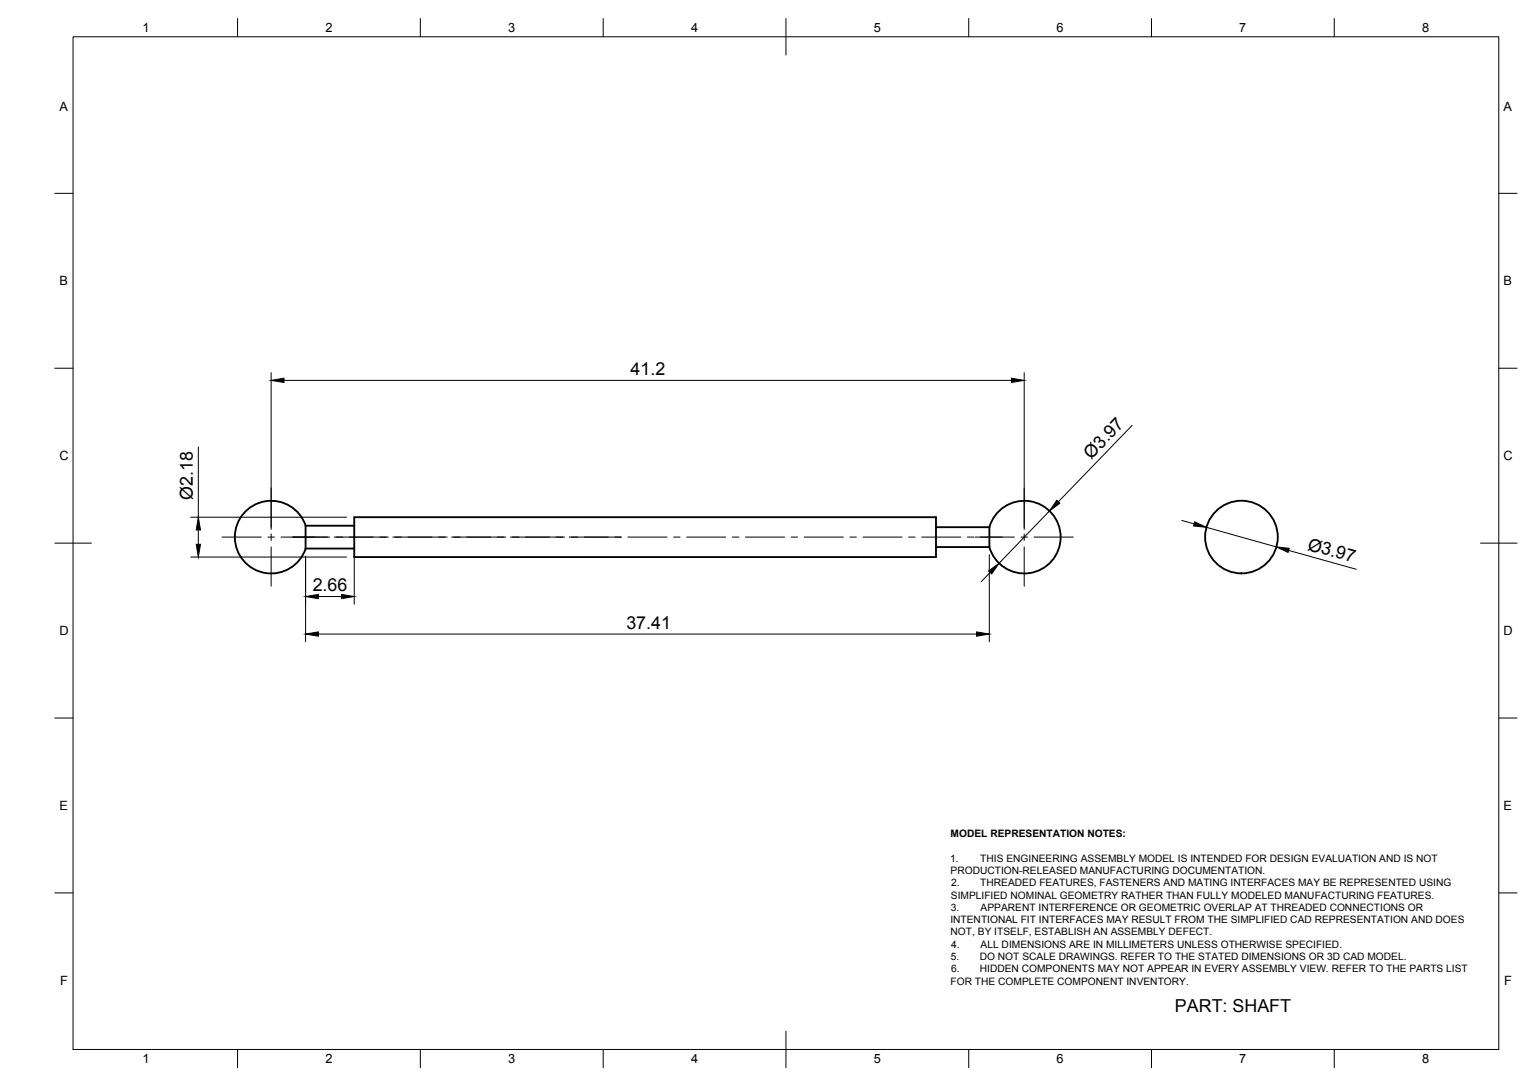
ISO-10303-21;
HEADER;
/* Generated by software containing ST-Developer
 * from STEP Tools, Inc. (www.steptools.com) 
 */

FILE_DESCRIPTION(
/* description */ (''),
/* implementation_level */ '2;1');

FILE_NAME(
/* name */ 'Shaft.step',
/* time_stamp */ '2026-10-04T22:56:18-07:00',
/* author */ (''),
/* organization */ (''),
/* preprocessor_version */ 'ST-DEVELOPER v20.2',
/* originating_system */ 'Autodesk Translation Framework v15.15.0.0',
/* authorisation */ '');

FILE_SCHEMA (('AUTOMOTIVE_DESIGN { 1 0 10303 214 3 1 1 }'));
ENDSEC;

DATA;
#10=MECHANICAL_DESIGN_GEOMETRIC_PRESENTATION_REPRESENTATION('',(#192),#14544);
#169=SPHERICAL_SURFACE('',#1978,1.9854168202488);
#170=SPHERICAL_SURFACE('',#1980,1.9854168202488);
#176=SHAPE_REPRESENTATION_RELATIONSHIP('SRR','None',#14578,#184);
#184=ADVANCED_BREP_SHAPE_REPRESENTATION('',(#200),#14538);
#192=STYLED_ITEM('',(#14627),#200);
#200=MANIFOLD_SOLID_BREP('Body1',#1828);
#215=LINE('',#2670,#271);
#216=LINE('',#2678,#272);
#217=LINE('',#2685,#273);
#271=VECTOR('',#2229,0.544851764215984);
#272=VECTOR('',#2240,1.08970352843197);
#273=VECTOR('',#2249,0.625182919763592);
#327=CYLINDRICAL_SURFACE('',#1967,0.544851764215984);
#328=CYLINDRICAL_SURFACE('',#1972,1.08970352843197);
#329=CYLINDRICAL_SURFACE('',#1976,0.625182919763592);
#378=FACE_BOUND('',#534,.T.);
#379=FACE_BOUND('',#537,.T.);
#419=FACE_OUTER_BOUND('',#532,.T.);
#420=FACE_OUTER_BOUND('',#533,.T.);
#421=FACE_OUTER_BOUND('',#535,.T.);
#422=FACE_OUTER_BOUND('',#536,.T.);
#423=FACE_OUTER_BOUND('',#538,.T.);
#424=FACE_OUTER_BOUND('',#539,.T.);
#425=FACE_OUTER_BOUND('',#540,.T.);
#532=EDGE_LOOP('',(#1229,#1230,#1231,#1232));
#533=EDGE_LOOP('',(#1233));
#534=EDGE_LOOP('',(#1234));
#535=EDGE_LOOP('',(#1235,#1236,#1237,#1238));
#536=EDGE_LOOP('',(#1239));
#537=EDGE_LOOP('',(#1240));
#538=EDGE_LOOP('',(#1241,#1242,#1243,#1244));
#539=EDGE_LOOP('',(#1245,#1246,#1247));
#540=EDGE_LOOP('',(#1248,#1249,#1250));
#658=CIRCLE('',#1968,0.544851764215984);
#659=CIRCLE('',#1969,0.544851764215984);
#660=CIRCLE('',#1971,1.08970352843197);
#661=CIRCLE('',#1973,1.08970352843197);
#662=CIRCLE('',#1975,0.625182919763592);
#663=CIRCLE('',#1977,0.625182919763592);
#664=CIRCLE('',#1979,1.9854168202488);
#665=CIRCLE('',#1981,1.9854168202488);
#744=VERTEX_POINT('',#2667);
#745=VERTEX_POINT('',#2669);
#746=VERTEX_POINT('',#2673);
#747=VERTEX_POINT('',#2676);
#748=VERTEX_POINT('',#2680);
#749=VERTEX_POINT('',#2683);
#750=VERTEX_POINT('',#2687);
#751=VERTEX_POINT('',#2690);
#943=EDGE_CURVE('',#744,#744,#658,.T.);
#944=EDGE_CURVE('',#744,#745,#215,.T.);
#945=EDGE_CURVE('',#745,#745,#659,.T.);
#946=EDGE_CURVE('',#746,#746,#660,.T.);
#947=EDGE_CURVE('',#747,#747,#661,.T.);
#948=EDGE_CURVE('',#747,#746,#216,.T.);
#949=EDGE_CURVE('',#748,#748,#662,.T.);
#950=EDGE_CURVE('',#749,#749,#663,.T.);
#951=EDGE_CURVE('',#749,#748,#217,.T.);
#952=EDGE_CURVE('',#750,#749,#664,.T.);
#953=EDGE_CURVE('',#745,#751,#665,.T.);
#1229=ORIENTED_EDGE('',*,*,#943,.F.);
#1230=ORIENTED_EDGE('',*,*,#944,.T.);
#1231=ORIENTED_EDGE('',*,*,#945,.T.);
#1232=ORIENTED_EDGE('',*,*,#944,.F.);
#1233=ORIENTED_EDGE('',*,*,#946,.F.);
#1234=ORIENTED_EDGE('',*,*,#943,.T.);
#1235=ORIENTED_EDGE('',*,*,#947,.F.);
#1236=ORIENTED_EDGE('',*,*,#948,.T.);
#1237=ORIENTED_EDGE('',*,*,#946,.T.);
#1238=ORIENTED_EDGE('',*,*,#948,.F.);
#1239=ORIENTED_EDGE('',*,*,#947,.T.);
#1240=ORIENTED_EDGE('',*,*,#949,.F.);
#1241=ORIENTED_EDGE('',*,*,#950,.F.);
#1242=ORIENTED_EDGE('',*,*,#951,.T.);
#1243=ORIENTED_EDGE('',*,*,#949,.T.);
#1244=ORIENTED_EDGE('',*,*,#951,.F.);
#1245=ORIENTED_EDGE('',*,*,#950,.T.);
#1246=ORIENTED_EDGE('',*,*,#952,.F.);
#1247=ORIENTED_EDGE('',*,*,#952,.T.);
#1248=ORIENTED_EDGE('',*,*,#945,.F.);
#1249=ORIENTED_EDGE('',*,*,#953,.T.);
#1250=ORIENTED_EDGE('',*,*,#953,.F.);
#1695=PLANE('',#1970);
#1696=PLANE('',#1974);
#1741=ADVANCED_FACE('',(#419),#327,.T.);
#1742=ADVANCED_FACE('',(#420,#378),#1695,.T.);
#1743=ADVANCED_FACE('',(#421),#328,.T.);
#1744=ADVANCED_FACE('',(#422,#379),#1696,.T.);
#1745=ADVANCED_FACE('',(#423),#329,.T.);
#1746=ADVANCED_FACE('',(#424),#169,.T.);
#1747=ADVANCED_FACE('',(#425),#170,.T.);
#1828=CLOSED_SHELL('',(#1741,#1742,#1743,#1744,#1745,#1746,#1747));
#1966=AXIS2_PLACEMENT_3D('',#2665,#2223,#2224);
#1967=AXIS2_PLACEMENT_3D('',#2666,#2225,#2226);
#1968=AXIS2_PLACEMENT_3D('',#2668,#2227,#2228);
#1969=AXIS2_PLACEMENT_3D('',#2671,#2230,#2231);
#1970=AXIS2_PLACEMENT_3D('',#2672,#2232,#2233);
#1971=AXIS2_PLACEMENT_3D('',#2674,#2234,#2235);
#1972=AXIS2_PLACEMENT_3D('',#2675,#2236,#2237);
#1973=AXIS2_PLACEMENT_3D('',#2677,#2238,#2239);
#1974=AXIS2_PLACEMENT_3D('',#2679,#2241,#2242);
#1975=AXIS2_PLACEMENT_3D('',#2681,#2243,#2244);
#1976=AXIS2_PLACEMENT_3D('',#2682,#2245,#2246);
#1977=AXIS2_PLACEMENT_3D('',#2684,#2247,#2248);
#1978=AXIS2_PLACEMENT_3D('',#2686,#2250,#2251);
#1979=AXIS2_PLACEMENT_3D('',#2688,#2252,#2253);
#1980=AXIS2_PLACEMENT_3D('',#2689,#2254,#2255);
#1981=AXIS2_PLACEMENT_3D('',#2691,#2256,#2257);
#2223=DIRECTION('axis',(0.,0.,1.));
#2224=DIRECTION('refdir',(1.,0.,0.));
#2225=DIRECTION('center_axis',(0.,0.,1.));
#2226=DIRECTION('ref_axis',(1.,0.,0.));
#2227=DIRECTION('center_axis',(0.,0.,1.));
#2228=DIRECTION('ref_axis',(1.,0.,0.));
#2229=DIRECTION('',(0.,0.,-1.));
#2230=DIRECTION('center_axis',(0.,0.,1.));
#2231=DIRECTION('ref_axis',(1.,0.,0.));
#2232=DIRECTION('center_axis',(0.,0.,-1.));
#2233=DIRECTION('ref_axis',(-1.,0.,0.));
#2234=DIRECTION('center_axis',(0.,0.,1.));
#2235=DIRECTION('ref_axis',(1.,0.,0.));
#2236=DIRECTION('center_axis',(0.,0.,1.));
#2237=DIRECTION('ref_axis',(1.,0.,0.));
#2238=DIRECTION('center_axis',(0.,0.,1.));
#2239=DIRECTION('ref_axis',(1.,0.,0.));
#2240=DIRECTION('',(0.,0.,-1.));
#2241=DIRECTION('center_axis',(0.,0.,1.));
#2242=DIRECTION('ref_axis',(1.,0.,0.));
#2243=DIRECTION('center_axis',(0.,0.,1.));
#2244=DIRECTION('ref_axis',(1.,0.,0.));
#2245=DIRECTION('center_axis',(0.,0.,1.));
#2246=DIRECTION('ref_axis',(1.,0.,0.));
#2247=DIRECTION('center_axis',(0.,0.,1.));
#2248=DIRECTION('ref_axis',(1.,0.,0.));
#2249=DIRECTION('',(0.,0.,-1.));
#2250=DIRECTION('center_axis',(1.22464679914735E-16,0.,1.));
#2251=DIRECTION('ref_axis',(1.,0.,0.));
#2252=DIRECTION('center_axis',(1.22464679914735E-16,-1.,-7.49879891330929E-33));
#2253=DIRECTION('ref_axis',(-1.,-1.22464679914735E-16,0.));
#2254=DIRECTION('center_axis',(1.22464679914735E-16,0.,1.));
#2255=DIRECTION('ref_axis',(1.,0.,0.));
#2256=DIRECTION('center_axis',(1.22464679914735E-16,-1.,-7.49879891330928E-33));
#2257=DIRECTION('ref_axis',(-1.,-1.22464679914735E-16,0.));
#2665=CARTESIAN_POINT('',(0.,0.,0.));
#2666=CARTESIAN_POINT('Origin',(0.,0.,14.8197830204816));
#2667=CARTESIAN_POINT('',(-0.544851764215984,-6.67250969056894E-17,16.2795718072011));
#2668=CARTESIAN_POINT('Origin',(0.,0.,16.2795718072011));
#2669=CARTESIAN_POINT('',(-0.544851764215984,-6.67250969056894E-17,13.3599942337622));
#2670=CARTESIAN_POINT('',(-0.544851764215984,-6.67250969056893E-17,14.8197830204816));
#2671=CARTESIAN_POINT('Origin',(0.,0.,13.3599942337622));
#2672=CARTESIAN_POINT('Origin',(1.08970352843197,0.,16.2795718072011));
#2673=CARTESIAN_POINT('',(-1.08970352843197,-1.33450193811379E-16,16.2795718072011));
#2674=CARTESIAN_POINT('Origin',(0.,0.,16.2795718072011));
#2675=CARTESIAN_POINT('Origin',(0.,0.,32.1916732743837));
#2676=CARTESIAN_POINT('',(-1.08970352843197,-1.33450193811379E-16,48.1037747415664));
#2677=CARTESIAN_POINT('Origin',(0.,0.,48.1037747415664));
#2678=CARTESIAN_POINT('',(-1.08970352843197,-1.33450193811379E-16,32.1916732743837));
#2679=CARTESIAN_POINT('Origin',(0.625182919763592,0.,48.1037747415664));
#2680=CARTESIAN_POINT('',(-0.625182919763592,-7.65628261570079E-17,48.1037747415664));
#2681=CARTESIAN_POINT('Origin',(0.,0.,48.1037747415664));
#2682=CARTESIAN_POINT('Origin',(0.,0.,49.4350798260675));
#2683=CARTESIAN_POINT('',(-0.625182919763592,-7.65628261570079E-17,50.7663849105686));
#2684=CARTESIAN_POINT('Origin',(0.,0.,50.7663849105686));
#2685=CARTESIAN_POINT('',(-0.625182919763592,-7.6562826157008E-17,49.4350798260675));
#2686=CARTESIAN_POINT('Origin',(0.,0.,52.6508016020046));
#2687=CARTESIAN_POINT('',(-1.2157171769455E-16,-2.97764829882954E-32,54.6362184222534));
#2688=CARTESIAN_POINT('Origin',(0.,0.,52.6508016020046));
#2689=CARTESIAN_POINT('Origin',(0.,0.,11.4508016020046));
#2690=CARTESIAN_POINT('',(-1.2157171769455E-16,-1.3684555315672E-47,9.4653847817558));
#2691=CARTESIAN_POINT('Origin',(0.,0.,11.4508016020046));
#14528=UNCERTAINTY_MEASURE_WITH_UNIT(LENGTH_MEASURE(0.01),#14545,
'DISTANCE_ACCURACY_VALUE',
'Maximum model space distance between geometric entities at asserted c
onnectivities');
#14534=UNCERTAINTY_MEASURE_WITH_UNIT(LENGTH_MEASURE(0.01),#14545,
'DISTANCE_ACCURACY_VALUE',
'Maximum model space distance between geometric entities at asserted c
onnectivities');
#14538=(
GEOMETRIC_REPRESENTATION_CONTEXT(3)
GLOBAL_UNCERTAINTY_ASSIGNED_CONTEXT((#14528))
GLOBAL_UNIT_ASSIGNED_CONTEXT((#14545,#14547,#14548))
REPRESENTATION_CONTEXT('','3D')
);
#14544=(
GEOMETRIC_REPRESENTATION_CONTEXT(3)
GLOBAL_UNCERTAINTY_ASSIGNED_CONTEXT((#14534))
GLOBAL_UNIT_ASSIGNED_CONTEXT((#14545,#14547,#14548))
REPRESENTATION_CONTEXT('','3D')
);
#14545=(
LENGTH_UNIT()
NAMED_UNIT(*)
SI_UNIT(.MILLI.,.METRE.)
);
#14547=(
NAMED_UNIT(*)
PLANE_ANGLE_UNIT()
SI_UNIT($,.RADIAN.)
);
#14548=(
NAMED_UNIT(*)
SI_UNIT($,.STERADIAN.)
SOLID_ANGLE_UNIT()
);
#14552=SHAPE_DEFINITION_REPRESENTATION(#14561,#14578);
#14561=PRODUCT_DEFINITION_SHAPE('',$,#14588);
#14578=SHAPE_REPRESENTATION('',(#1966),#14538);
#14584=PRODUCT_DEFINITION_CONTEXT('part definition',#14613,'design');
#14588=PRODUCT_DEFINITION('Shaft','Shaft',#14597,#14584);
#14597=PRODUCT_DEFINITION_FORMATION('',$,#14618);
#14613=APPLICATION_CONTEXT(
'Core Data for Automotive Mechanical Design Process');
#14614=PRODUCT_CONTEXT('part definition',#14613,'mechanical');
#14618=PRODUCT('Shaft','Shaft',$,(#14614));
#14627=PRESENTATION_STYLE_ASSIGNMENT((#14631));
#14631=SURFACE_STYLE_USAGE(.BOTH.,#14635);
#14635=SURFACE_SIDE_STYLE('',(#14639));
#14639=SURFACE_STYLE_FILL_AREA(#14643);
#14643=FILL_AREA_STYLE('Opaque(203,203,203)',(#14647));
#14647=FILL_AREA_STYLE_COLOUR('Opaque(203,203,203)',#14651);
#14651=COLOUR_RGB('Opaque(203,203,203)', 0.31764706, 0.68627451, 0.89019608);
ENDSEC;
END-ISO-10303-21;
